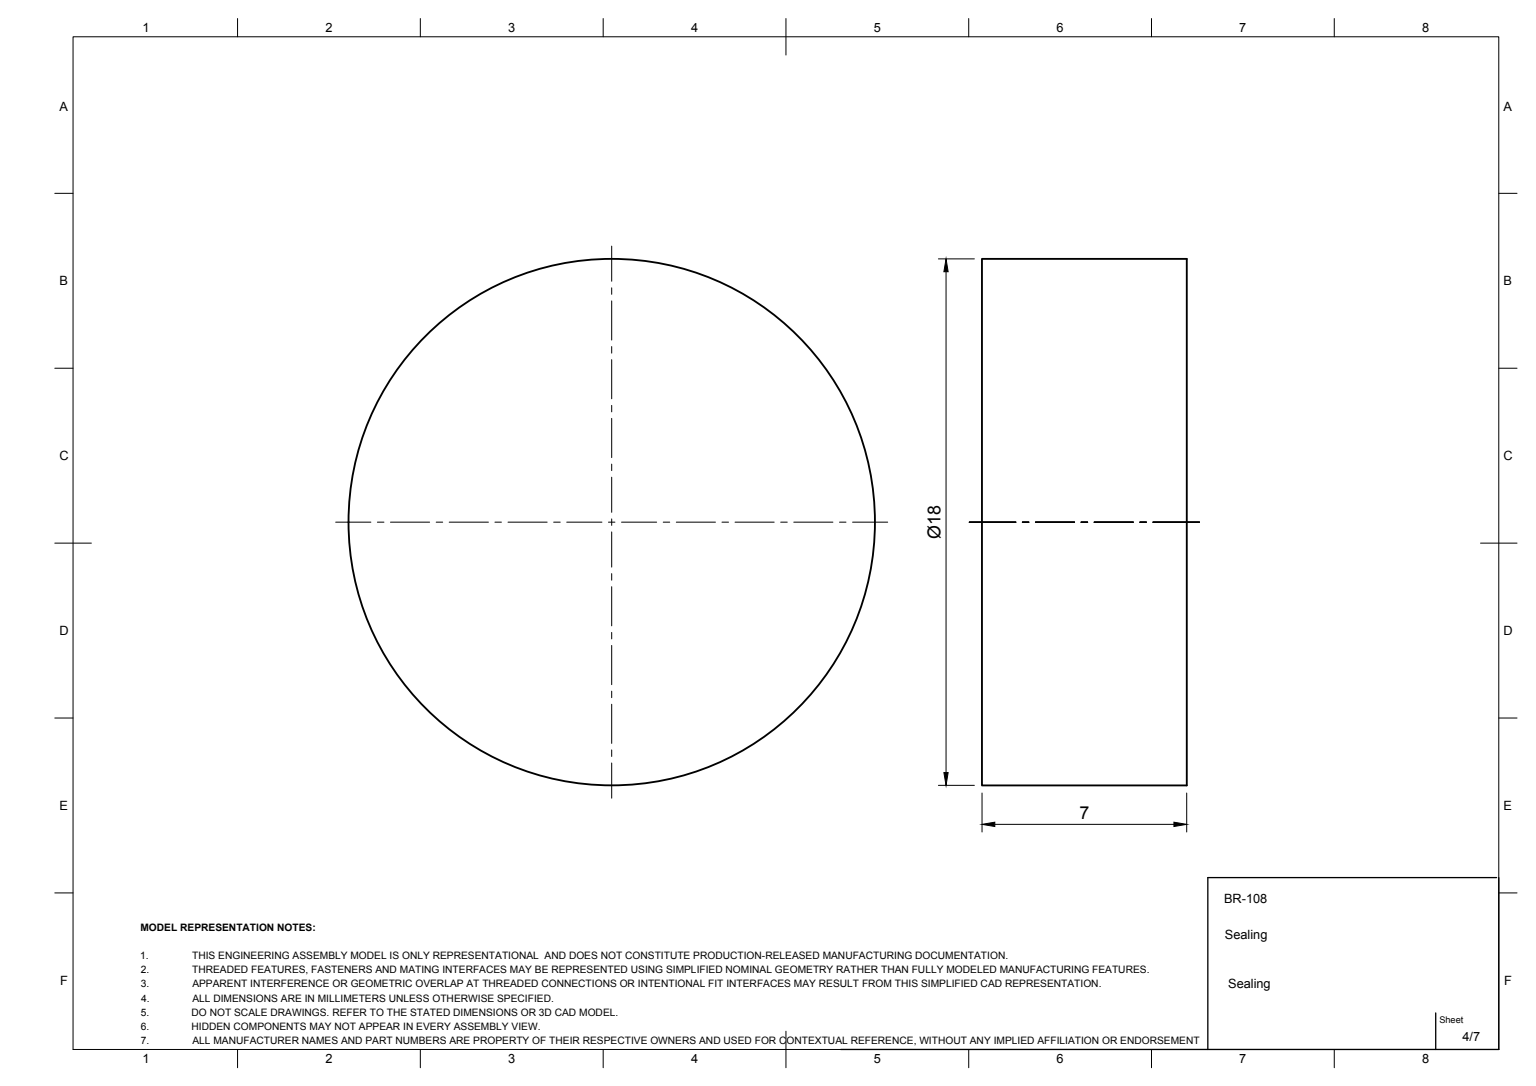
ISO-10303-21;
HEADER;
/* Generated by software containing ST-Developer
 * from STEP Tools, Inc. (www.steptools.com) 
 */

FILE_DESCRIPTION(
/* description */ (''),
/* implementation_level */ '2;1');

FILE_NAME(
/* name */ 'Sealing.step',
/* time_stamp */ '2026-11-14T03:52:36-08:00',
/* author */ (''),
/* organization */ (''),
/* preprocessor_version */ 'ST-DEVELOPER v20.2',
/* originating_system */ 'Autodesk Translation Framework v15.17.0.0',
/* authorisation */ '');

FILE_SCHEMA (('AUTOMOTIVE_DESIGN { 1 0 10303 214 3 1 1 }'));
ENDSEC;

DATA;
#10=MECHANICAL_DESIGN_GEOMETRIC_PRESENTATION_REPRESENTATION('',(#192),#19443);
#176=SHAPE_REPRESENTATION_RELATIONSHIP('SRR','None',#19476,#184);
#184=ADVANCED_BREP_SHAPE_REPRESENTATION('',(#200),#19436);
#192=STYLED_ITEM('',(#19524),#200);
#200=MANIFOLD_SOLID_BREP('Body1',#2019);
#222=PLANE('',#2129);
#223=PLANE('',#2130);
#277=FACE_OUTER_BOUND('',#375,.T.);
#278=FACE_OUTER_BOUND('',#376,.T.);
#279=FACE_OUTER_BOUND('',#377,.T.);
#375=EDGE_LOOP('',(#1303,#1304,#1305,#1306));
#376=EDGE_LOOP('',(#1307));
#377=EDGE_LOOP('',(#1308));
#480=LINE('',#2716,#607);
#607=VECTOR('',#2294,9.);
#736=CIRCLE('',#2127,9.);
#737=CIRCLE('',#2128,9.);
#780=VERTEX_POINT('',#2713);
#781=VERTEX_POINT('',#2715);
#1000=EDGE_CURVE('',#780,#780,#736,.T.);
#1001=EDGE_CURVE('',#780,#781,#480,.T.);
#1002=EDGE_CURVE('',#781,#781,#737,.T.);
#1303=ORIENTED_EDGE('',*,*,#1000,.F.);
#1304=ORIENTED_EDGE('',*,*,#1001,.T.);
#1305=ORIENTED_EDGE('',*,*,#1002,.T.);
#1306=ORIENTED_EDGE('',*,*,#1001,.F.);
#1307=ORIENTED_EDGE('',*,*,#1000,.T.);
#1308=ORIENTED_EDGE('',*,*,#1002,.F.);
#1887=CYLINDRICAL_SURFACE('',#2126,9.);
#1926=ADVANCED_FACE('',(#277),#1887,.T.);
#1927=ADVANCED_FACE('',(#278),#222,.T.);
#1928=ADVANCED_FACE('',(#279),#223,.F.);
#2019=CLOSED_SHELL('',(#1926,#1927,#1928));
#2125=AXIS2_PLACEMENT_3D('',#2711,#2288,#2289);
#2126=AXIS2_PLACEMENT_3D('',#2712,#2290,#2291);
#2127=AXIS2_PLACEMENT_3D('',#2714,#2292,#2293);
#2128=AXIS2_PLACEMENT_3D('',#2717,#2295,#2296);
#2129=AXIS2_PLACEMENT_3D('',#2718,#2297,#2298);
#2130=AXIS2_PLACEMENT_3D('',#2719,#2299,#2300);
#2288=DIRECTION('axis',(0.,0.,1.));
#2289=DIRECTION('refdir',(1.,0.,0.));
#2290=DIRECTION('center_axis',(0.,0.,1.));
#2291=DIRECTION('ref_axis',(-1.,0.,0.));
#2292=DIRECTION('center_axis',(0.,0.,1.));
#2293=DIRECTION('ref_axis',(-1.,0.,0.));
#2294=DIRECTION('',(0.,0.,-1.));
#2295=DIRECTION('center_axis',(0.,0.,1.));
#2296=DIRECTION('ref_axis',(-1.,0.,0.));
#2297=DIRECTION('center_axis',(0.,0.,1.));
#2298=DIRECTION('ref_axis',(-1.,0.,0.));
#2299=DIRECTION('center_axis',(0.,0.,1.));
#2300=DIRECTION('ref_axis',(-1.,0.,0.));
#2711=CARTESIAN_POINT('',(0.,0.,0.));
#2712=CARTESIAN_POINT('Origin',(0.,0.,170.));
#2713=CARTESIAN_POINT('',(9.,1.10218211923262E-15,177.));
#2714=CARTESIAN_POINT('Origin',(0.,0.,177.));
#2715=CARTESIAN_POINT('',(9.,1.10218211923262E-15,170.));
#2716=CARTESIAN_POINT('',(9.,1.10218211923262E-15,170.));
#2717=CARTESIAN_POINT('Origin',(0.,0.,170.));
#2718=CARTESIAN_POINT('Origin',(0.,0.,177.));
#2719=CARTESIAN_POINT('Origin',(0.,0.,170.));
#19426=UNCERTAINTY_MEASURE_WITH_UNIT(LENGTH_MEASURE(0.01),#19444,
'DISTANCE_ACCURACY_VALUE',
'Maximum model space distance between geometric entities at asserted c
onnectivities');
#19433=UNCERTAINTY_MEASURE_WITH_UNIT(LENGTH_MEASURE(0.01),#19444,
'DISTANCE_ACCURACY_VALUE',
'Maximum model space distance between geometric entities at asserted c
onnectivities');
#19436=(
GEOMETRIC_REPRESENTATION_CONTEXT(3)
GLOBAL_UNCERTAINTY_ASSIGNED_CONTEXT((#19426))
GLOBAL_UNIT_ASSIGNED_CONTEXT((#19444,#19446,#19447))
REPRESENTATION_CONTEXT('','3D')
);
#19443=(
GEOMETRIC_REPRESENTATION_CONTEXT(3)
GLOBAL_UNCERTAINTY_ASSIGNED_CONTEXT((#19433))
GLOBAL_UNIT_ASSIGNED_CONTEXT((#19444,#19446,#19447))
REPRESENTATION_CONTEXT('','3D')
);
#19444=(
LENGTH_UNIT()
NAMED_UNIT(*)
SI_UNIT(.MILLI.,.METRE.)
);
#19446=(
NAMED_UNIT(*)
PLANE_ANGLE_UNIT()
SI_UNIT($,.RADIAN.)
);
#19447=(
NAMED_UNIT(*)
SI_UNIT($,.STERADIAN.)
SOLID_ANGLE_UNIT()
);
#19450=SHAPE_DEFINITION_REPRESENTATION(#19459,#19476);
#19459=PRODUCT_DEFINITION_SHAPE('',$,#19486);
#19476=SHAPE_REPRESENTATION('',(#2125),#19436);
#19483=PRODUCT_DEFINITION_CONTEXT('part definition',#19512,'design');
#19486=PRODUCT_DEFINITION('Sealing','Sealing',#19495,#19483);
#19495=PRODUCT_DEFINITION_FORMATION('',$,#19516);
#19512=APPLICATION_CONTEXT(
'Core Data for Automotive Mechanical Design Process');
#19513=PRODUCT_CONTEXT('part definition',#19512,'mechanical');
#19516=PRODUCT('Sealing','Sealing',$,(#19513));
#19524=PRESENTATION_STYLE_ASSIGNMENT((#19527));
#19527=SURFACE_STYLE_USAGE(.BOTH.,#19530);
#19530=SURFACE_SIDE_STYLE('',(#19533));
#19533=SURFACE_STYLE_FILL_AREA(#19536);
#19536=FILL_AREA_STYLE('Opaque(36,31,37)',(#19539));
#19539=FILL_AREA_STYLE_COLOUR('Opaque(36,31,37)',#19542);
#19542=COLOUR_RGB('Opaque(36,31,37)',0.141176470588235,0.12156862745098,
0.145098039215686);
ENDSEC;
END-ISO-10303-21;
